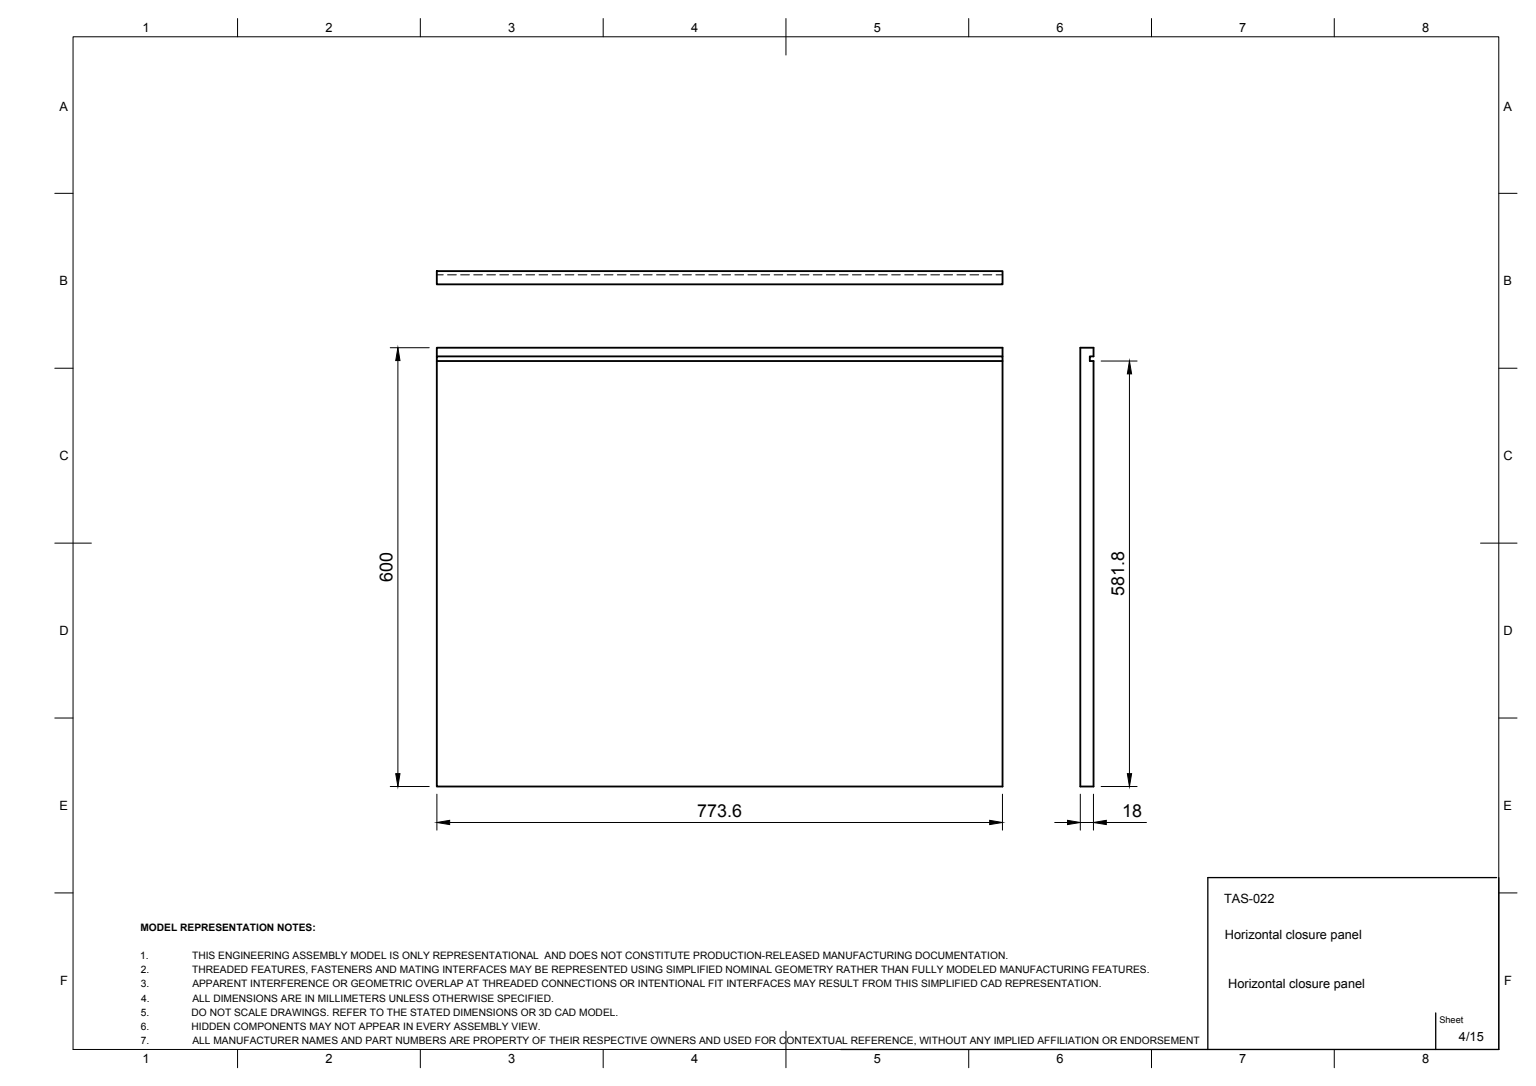
ISO-10303-21;
HEADER;
/* Generated by software containing ST-Developer
 * from STEP Tools, Inc. (www.steptools.com) 
 */

FILE_DESCRIPTION(
/* description */ (''),
/* implementation_level */ '2;1');

FILE_NAME(
/* name */ 'Horizontal closure panel.step',
/* time_stamp */ '2026-11-15T21:02:08-08:00',
/* author */ (''),
/* organization */ (''),
/* preprocessor_version */ 'ST-DEVELOPER v20.2',
/* originating_system */ 'Autodesk Translation Framework v15.17.0.0',
/* authorisation */ '');

FILE_SCHEMA (('AUTOMOTIVE_DESIGN { 1 0 10303 214 3 1 1 }'));
ENDSEC;

DATA;
#10=MECHANICAL_DESIGN_GEOMETRIC_PRESENTATION_REPRESENTATION('',(#609),#31566);
#579=SHAPE_REPRESENTATION_RELATIONSHIP('SRR','None',#31643,#594);
#594=ADVANCED_BREP_SHAPE_REPRESENTATION('',(#624),#31558);
#609=STYLED_ITEM('',(#31724),#624);
#624=MANIFOLD_SOLID_BREP('Body1',#5722);
#745=FACE_OUTER_BOUND('',#1042,.T.);
#746=FACE_OUTER_BOUND('',#1043,.T.);
#747=FACE_OUTER_BOUND('',#1044,.T.);
#748=FACE_OUTER_BOUND('',#1045,.T.);
#749=FACE_OUTER_BOUND('',#1046,.T.);
#750=FACE_OUTER_BOUND('',#1047,.T.);
#751=FACE_OUTER_BOUND('',#1048,.T.);
#752=FACE_OUTER_BOUND('',#1049,.T.);
#753=FACE_OUTER_BOUND('',#1050,.T.);
#754=FACE_OUTER_BOUND('',#1051,.T.);
#1042=EDGE_LOOP('',(#4197,#4198,#4199,#4200));
#1043=EDGE_LOOP('',(#4201,#4202,#4203,#4204));
#1044=EDGE_LOOP('',(#4205,#4206,#4207,#4208));
#1045=EDGE_LOOP('',(#4209,#4210,#4211,#4212,#4213,#4214,#4215,#4216));
#1046=EDGE_LOOP('',(#4217,#4218,#4219,#4220));
#1047=EDGE_LOOP('',(#4221,#4222,#4223,#4224));
#1048=EDGE_LOOP('',(#4225,#4226,#4227,#4228));
#1049=EDGE_LOOP('',(#4229,#4230,#4231,#4232,#4233,#4234,#4235,#4236));
#1050=EDGE_LOOP('',(#4237,#4238,#4239,#4240));
#1051=EDGE_LOOP('',(#4241,#4242,#4243,#4244));
#1439=LINE('',#8161,#1946);
#1440=LINE('',#8163,#1947);
#1441=LINE('',#8165,#1948);
#1442=LINE('',#8166,#1949);
#1443=LINE('',#8170,#1950);
#1444=LINE('',#8172,#1951);
#1445=LINE('',#8174,#1952);
#1446=LINE('',#8175,#1953);
#1447=LINE('',#8177,#1954);
#1448=LINE('',#8178,#1955);
#1449=LINE('',#8181,#1956);
#1450=LINE('',#8183,#1957);
#1451=LINE('',#8185,#1958);
#1452=LINE('',#8187,#1959);
#1453=LINE('',#8188,#1960);
#1454=LINE('',#8191,#1961);
#1455=LINE('',#8192,#1962);
#1456=LINE('',#8195,#1963);
#1457=LINE('',#8197,#1964);
#1458=LINE('',#8198,#1965);
#1459=LINE('',#8201,#1966);
#1460=LINE('',#8202,#1967);
#1461=LINE('',#8204,#1968);
#1462=LINE('',#8205,#1969);
#1946=VECTOR('',#6865,1.);
#1947=VECTOR('',#6866,1.);
#1948=VECTOR('',#6867,1.);
#1949=VECTOR('',#6868,1.);
#1950=VECTOR('',#6871,1.);
#1951=VECTOR('',#6872,1.);
#1952=VECTOR('',#6873,1.);
#1953=VECTOR('',#6874,1.);
#1954=VECTOR('',#6877,1.);
#1955=VECTOR('',#6878,1.);
#1956=VECTOR('',#6881,1.);
#1957=VECTOR('',#6882,1.);
#1958=VECTOR('',#6883,1.);
#1959=VECTOR('',#6884,1.);
#1960=VECTOR('',#6885,1.);
#1961=VECTOR('',#6888,1.);
#1962=VECTOR('',#6889,1.);
#1963=VECTOR('',#6892,1.);
#1964=VECTOR('',#6893,1.);
#1965=VECTOR('',#6894,1.);
#1966=VECTOR('',#6897,1.);
#1967=VECTOR('',#6898,1.);
#1968=VECTOR('',#6901,1.);
#1969=VECTOR('',#6902,1.);
#2410=VERTEX_POINT('',#8159);
#2411=VERTEX_POINT('',#8160);
#2412=VERTEX_POINT('',#8162);
#2413=VERTEX_POINT('',#8164);
#2414=VERTEX_POINT('',#8168);
#2415=VERTEX_POINT('',#8169);
#2416=VERTEX_POINT('',#8171);
#2417=VERTEX_POINT('',#8173);
#2418=VERTEX_POINT('',#8180);
#2419=VERTEX_POINT('',#8182);
#2420=VERTEX_POINT('',#8184);
#2421=VERTEX_POINT('',#8186);
#2422=VERTEX_POINT('',#8190);
#2423=VERTEX_POINT('',#8194);
#2424=VERTEX_POINT('',#8196);
#2425=VERTEX_POINT('',#8200);
#3094=EDGE_CURVE('',#2410,#2411,#1439,.T.);
#3095=EDGE_CURVE('',#2412,#2410,#1440,.T.);
#3096=EDGE_CURVE('',#2413,#2412,#1441,.T.);
#3097=EDGE_CURVE('',#2411,#2413,#1442,.T.);
#3098=EDGE_CURVE('',#2414,#2415,#1443,.T.);
#3099=EDGE_CURVE('',#2416,#2414,#1444,.T.);
#3100=EDGE_CURVE('',#2417,#2416,#1445,.T.);
#3101=EDGE_CURVE('',#2415,#2417,#1446,.T.);
#3102=EDGE_CURVE('',#2413,#2416,#1447,.T.);
#3103=EDGE_CURVE('',#2417,#2412,#1448,.T.);
#3104=EDGE_CURVE('',#2418,#2410,#1449,.T.);
#3105=EDGE_CURVE('',#2419,#2418,#1450,.T.);
#3106=EDGE_CURVE('',#2419,#2420,#1451,.T.);
#3107=EDGE_CURVE('',#2420,#2421,#1452,.T.);
#3108=EDGE_CURVE('',#2415,#2421,#1453,.T.);
#3109=EDGE_CURVE('',#2411,#2422,#1454,.T.);
#3110=EDGE_CURVE('',#2422,#2418,#1455,.T.);
#3111=EDGE_CURVE('',#2420,#2423,#1456,.T.);
#3112=EDGE_CURVE('',#2423,#2424,#1457,.T.);
#3113=EDGE_CURVE('',#2421,#2424,#1458,.T.);
#3114=EDGE_CURVE('',#2425,#2419,#1459,.T.);
#3115=EDGE_CURVE('',#2425,#2422,#1460,.T.);
#3116=EDGE_CURVE('',#2424,#2414,#1461,.T.);
#3117=EDGE_CURVE('',#2423,#2425,#1462,.T.);
#4197=ORIENTED_EDGE('',*,*,#3094,.F.);
#4198=ORIENTED_EDGE('',*,*,#3095,.F.);
#4199=ORIENTED_EDGE('',*,*,#3096,.F.);
#4200=ORIENTED_EDGE('',*,*,#3097,.F.);
#4201=ORIENTED_EDGE('',*,*,#3098,.F.);
#4202=ORIENTED_EDGE('',*,*,#3099,.F.);
#4203=ORIENTED_EDGE('',*,*,#3100,.F.);
#4204=ORIENTED_EDGE('',*,*,#3101,.F.);
#4205=ORIENTED_EDGE('',*,*,#3102,.F.);
#4206=ORIENTED_EDGE('',*,*,#3096,.T.);
#4207=ORIENTED_EDGE('',*,*,#3103,.F.);
#4208=ORIENTED_EDGE('',*,*,#3100,.T.);
#4209=ORIENTED_EDGE('',*,*,#3101,.T.);
#4210=ORIENTED_EDGE('',*,*,#3103,.T.);
#4211=ORIENTED_EDGE('',*,*,#3095,.T.);
#4212=ORIENTED_EDGE('',*,*,#3104,.F.);
#4213=ORIENTED_EDGE('',*,*,#3105,.F.);
#4214=ORIENTED_EDGE('',*,*,#3106,.T.);
#4215=ORIENTED_EDGE('',*,*,#3107,.T.);
#4216=ORIENTED_EDGE('',*,*,#3108,.F.);
#4217=ORIENTED_EDGE('',*,*,#3094,.T.);
#4218=ORIENTED_EDGE('',*,*,#3109,.T.);
#4219=ORIENTED_EDGE('',*,*,#3110,.T.);
#4220=ORIENTED_EDGE('',*,*,#3104,.T.);
#4221=ORIENTED_EDGE('',*,*,#3111,.T.);
#4222=ORIENTED_EDGE('',*,*,#3112,.T.);
#4223=ORIENTED_EDGE('',*,*,#3113,.F.);
#4224=ORIENTED_EDGE('',*,*,#3107,.F.);
#4225=ORIENTED_EDGE('',*,*,#3114,.T.);
#4226=ORIENTED_EDGE('',*,*,#3105,.T.);
#4227=ORIENTED_EDGE('',*,*,#3110,.F.);
#4228=ORIENTED_EDGE('',*,*,#3115,.F.);
#4229=ORIENTED_EDGE('',*,*,#3099,.T.);
#4230=ORIENTED_EDGE('',*,*,#3116,.F.);
#4231=ORIENTED_EDGE('',*,*,#3112,.F.);
#4232=ORIENTED_EDGE('',*,*,#3117,.T.);
#4233=ORIENTED_EDGE('',*,*,#3115,.T.);
#4234=ORIENTED_EDGE('',*,*,#3109,.F.);
#4235=ORIENTED_EDGE('',*,*,#3097,.T.);
#4236=ORIENTED_EDGE('',*,*,#3102,.T.);
#4237=ORIENTED_EDGE('',*,*,#3098,.T.);
#4238=ORIENTED_EDGE('',*,*,#3108,.T.);
#4239=ORIENTED_EDGE('',*,*,#3113,.T.);
#4240=ORIENTED_EDGE('',*,*,#3116,.T.);
#4241=ORIENTED_EDGE('',*,*,#3117,.F.);
#4242=ORIENTED_EDGE('',*,*,#3111,.F.);
#4243=ORIENTED_EDGE('',*,*,#3106,.F.);
#4244=ORIENTED_EDGE('',*,*,#3114,.F.);
#5350=PLANE('',#6070);
#5351=PLANE('',#6071);
#5352=PLANE('',#6072);
#5353=PLANE('',#6073);
#5354=PLANE('',#6074);
#5355=PLANE('',#6075);
#5356=PLANE('',#6076);
#5357=PLANE('',#6077);
#5358=PLANE('',#6078);
#5359=PLANE('',#6079);
#5559=ADVANCED_FACE('',(#745),#5350,.F.);
#5560=ADVANCED_FACE('',(#746),#5351,.F.);
#5561=ADVANCED_FACE('',(#747),#5352,.T.);
#5562=ADVANCED_FACE('',(#748),#5353,.T.);
#5563=ADVANCED_FACE('',(#749),#5354,.T.);
#5564=ADVANCED_FACE('',(#750),#5355,.T.);
#5565=ADVANCED_FACE('',(#751),#5356,.T.);
#5566=ADVANCED_FACE('',(#752),#5357,.T.);
#5567=ADVANCED_FACE('',(#753),#5358,.T.);
#5568=ADVANCED_FACE('',(#754),#5359,.F.);
#5722=CLOSED_SHELL('',(#5559,#5560,#5561,#5562,#5563,#5564,#5565,#5566,
#5567,#5568));
#6069=AXIS2_PLACEMENT_3D('',#8157,#6861,#6862);
#6070=AXIS2_PLACEMENT_3D('',#8158,#6863,#6864);
#6071=AXIS2_PLACEMENT_3D('',#8167,#6869,#6870);
#6072=AXIS2_PLACEMENT_3D('',#8176,#6875,#6876);
#6073=AXIS2_PLACEMENT_3D('',#8179,#6879,#6880);
#6074=AXIS2_PLACEMENT_3D('',#8189,#6886,#6887);
#6075=AXIS2_PLACEMENT_3D('',#8193,#6890,#6891);
#6076=AXIS2_PLACEMENT_3D('',#8199,#6895,#6896);
#6077=AXIS2_PLACEMENT_3D('',#8203,#6899,#6900);
#6078=AXIS2_PLACEMENT_3D('',#8206,#6903,#6904);
#6079=AXIS2_PLACEMENT_3D('',#8207,#6905,#6906);
#6861=DIRECTION('axis',(0.,0.,1.));
#6862=DIRECTION('refdir',(1.,0.,0.));
#6863=DIRECTION('center_axis',(0.,-1.,0.));
#6864=DIRECTION('ref_axis',(1.,0.,0.));
#6865=DIRECTION('',(-1.,0.,0.));
#6866=DIRECTION('',(0.,0.,1.));
#6867=DIRECTION('',(1.,0.,0.));
#6868=DIRECTION('',(0.,0.,-1.));
#6869=DIRECTION('center_axis',(0.,1.,0.));
#6870=DIRECTION('ref_axis',(-1.,0.,0.));
#6871=DIRECTION('',(1.,0.,0.));
#6872=DIRECTION('',(0.,0.,1.));
#6873=DIRECTION('',(-1.,0.,0.));
#6874=DIRECTION('',(0.,0.,-1.));
#6875=DIRECTION('center_axis',(0.,0.,1.));
#6876=DIRECTION('ref_axis',(1.,0.,0.));
#6877=DIRECTION('',(0.,1.,0.));
#6878=DIRECTION('',(0.,-1.,0.));
#6879=DIRECTION('center_axis',(1.,0.,0.));
#6880=DIRECTION('ref_axis',(0.,1.,0.));
#6881=DIRECTION('',(0.,1.,0.));
#6882=DIRECTION('',(0.,0.,1.));
#6883=DIRECTION('',(0.,1.,0.));
#6884=DIRECTION('',(0.,0.,1.));
#6885=DIRECTION('',(0.,1.,0.));
#6886=DIRECTION('center_axis',(0.,0.,1.));
#6887=DIRECTION('ref_axis',(1.,0.,0.));
#6888=DIRECTION('',(0.,-1.,0.));
#6889=DIRECTION('',(1.,0.,0.));
#6890=DIRECTION('center_axis',(0.,1.,0.));
#6891=DIRECTION('ref_axis',(-1.,0.,0.));
#6892=DIRECTION('',(-1.,0.,0.));
#6893=DIRECTION('',(0.,0.,1.));
#6894=DIRECTION('',(-1.,0.,0.));
#6895=DIRECTION('center_axis',(0.,-1.,0.));
#6896=DIRECTION('ref_axis',(1.,0.,0.));
#6897=DIRECTION('',(1.,0.,0.));
#6898=DIRECTION('',(0.,0.,1.));
#6899=DIRECTION('center_axis',(-1.,0.,0.));
#6900=DIRECTION('ref_axis',(0.,-1.,0.));
#6901=DIRECTION('',(0.,-1.,0.));
#6902=DIRECTION('',(0.,-1.,0.));
#6903=DIRECTION('center_axis',(0.,0.,1.));
#6904=DIRECTION('ref_axis',(1.,0.,0.));
#6905=DIRECTION('center_axis',(0.,0.,1.));
#6906=DIRECTION('ref_axis',(1.,0.,0.));
#8157=CARTESIAN_POINT('',(0.,0.,0.));
#8158=CARTESIAN_POINT('Origin',(0.,58.18,1.3));
#8159=CARTESIAN_POINT('',(77.36,58.18,1.8));
#8160=CARTESIAN_POINT('',(0.,58.18,1.8));
#8161=CARTESIAN_POINT('',(19.34,58.18,1.8));
#8162=CARTESIAN_POINT('',(77.36,58.18,1.3));
#8163=CARTESIAN_POINT('',(77.36,58.18,0.65));
#8164=CARTESIAN_POINT('',(0.,58.18,1.3));
#8165=CARTESIAN_POINT('',(0.,58.18,1.3));
#8166=CARTESIAN_POINT('',(0.,58.18,0.65));
#8167=CARTESIAN_POINT('Origin',(77.36,58.82,1.3));
#8168=CARTESIAN_POINT('',(0.,58.82,1.8));
#8169=CARTESIAN_POINT('',(77.36,58.82,1.8));
#8170=CARTESIAN_POINT('',(58.02,58.82,1.8));
#8171=CARTESIAN_POINT('',(0.,58.82,1.3));
#8172=CARTESIAN_POINT('',(0.,58.82,0.65));
#8173=CARTESIAN_POINT('',(77.36,58.82,1.3));
#8174=CARTESIAN_POINT('',(77.36,58.82,1.3));
#8175=CARTESIAN_POINT('',(77.36,58.82,0.65));
#8176=CARTESIAN_POINT('Origin',(38.68,58.5,1.3));
#8177=CARTESIAN_POINT('',(0.,59.25,1.3));
#8178=CARTESIAN_POINT('',(77.36,29.25,1.3));
#8179=CARTESIAN_POINT('Origin',(77.36,0.,0.));
#8180=CARTESIAN_POINT('',(77.36,0.,1.8));
#8181=CARTESIAN_POINT('',(77.36,0.,1.8));
#8182=CARTESIAN_POINT('',(77.36,0.,0.));
#8183=CARTESIAN_POINT('',(77.36,0.,0.));
#8184=CARTESIAN_POINT('',(77.36,60.,0.));
#8185=CARTESIAN_POINT('',(77.36,0.,0.));
#8186=CARTESIAN_POINT('',(77.36,60.,1.8));
#8187=CARTESIAN_POINT('',(77.36,60.,0.));
#8188=CARTESIAN_POINT('',(77.36,0.,1.8));
#8189=CARTESIAN_POINT('Origin',(38.68,30.,1.8));
#8190=CARTESIAN_POINT('',(0.,0.,1.8));
#8191=CARTESIAN_POINT('',(0.,60.,1.8));
#8192=CARTESIAN_POINT('',(0.,0.,1.8));
#8193=CARTESIAN_POINT('Origin',(77.36,60.,0.));
#8194=CARTESIAN_POINT('',(0.,60.,0.));
#8195=CARTESIAN_POINT('',(77.36,60.,0.));
#8196=CARTESIAN_POINT('',(0.,60.,1.8));
#8197=CARTESIAN_POINT('',(0.,60.,0.));
#8198=CARTESIAN_POINT('',(77.36,60.,1.8));
#8199=CARTESIAN_POINT('Origin',(0.,0.,0.));
#8200=CARTESIAN_POINT('',(0.,0.,0.));
#8201=CARTESIAN_POINT('',(0.,0.,0.));
#8202=CARTESIAN_POINT('',(0.,0.,0.));
#8203=CARTESIAN_POINT('Origin',(0.,60.,0.));
#8204=CARTESIAN_POINT('',(0.,60.,1.8));
#8205=CARTESIAN_POINT('',(0.,60.,0.));
#8206=CARTESIAN_POINT('Origin',(38.68,30.,1.8));
#8207=CARTESIAN_POINT('Origin',(38.68,30.,0.));
#31541=UNCERTAINTY_MEASURE_WITH_UNIT(LENGTH_MEASURE(0.001),#31567,
'DISTANCE_ACCURACY_VALUE',
'Maximum model space distance between geometric entities at asserted c
onnectivities');
#31549=UNCERTAINTY_MEASURE_WITH_UNIT(LENGTH_MEASURE(0.001),#31567,
'DISTANCE_ACCURACY_VALUE',
'Maximum model space distance between geometric entities at asserted c
onnectivities');
#31558=(
GEOMETRIC_REPRESENTATION_CONTEXT(3)
GLOBAL_UNCERTAINTY_ASSIGNED_CONTEXT((#31541))
GLOBAL_UNIT_ASSIGNED_CONTEXT((#31567,#31569,#31570))
REPRESENTATION_CONTEXT('','3D')
);
#31566=(
GEOMETRIC_REPRESENTATION_CONTEXT(3)
GLOBAL_UNCERTAINTY_ASSIGNED_CONTEXT((#31549))
GLOBAL_UNIT_ASSIGNED_CONTEXT((#31567,#31569,#31570))
REPRESENTATION_CONTEXT('','3D')
);
#31567=(
LENGTH_UNIT()
NAMED_UNIT(*)
SI_UNIT(.CENTI.,.METRE.)
);
#31569=(
NAMED_UNIT(*)
PLANE_ANGLE_UNIT()
SI_UNIT($,.RADIAN.)
);
#31570=(
NAMED_UNIT(*)
SI_UNIT($,.STERADIAN.)
SOLID_ANGLE_UNIT()
);
#31579=SHAPE_DEFINITION_REPRESENTATION(#31595,#31643);
#31595=PRODUCT_DEFINITION_SHAPE('',$,#31660);
#31643=SHAPE_REPRESENTATION('',(#6069),#31558);
#31651=PRODUCT_DEFINITION_CONTEXT('part definition',#31701,'design');
#31660=PRODUCT_DEFINITION('Horizontal closure panel',
'Horizontal closure panel',#31676,#31651);
#31676=PRODUCT_DEFINITION_FORMATION('',$,#31711);
#31701=APPLICATION_CONTEXT(
'Core Data for Automotive Mechanical Design Process');
#31702=PRODUCT_CONTEXT('part definition',#31701,'mechanical');
#31711=PRODUCT('Horizontal closure panel','Horizontal closure panel',$,
(#31702));
#31724=PRESENTATION_STYLE_ASSIGNMENT((#31731));
#31731=SURFACE_STYLE_USAGE(.BOTH.,#31738);
#31738=SURFACE_SIDE_STYLE('',(#31745));
#31745=SURFACE_STYLE_FILL_AREA(#31752);
#31752=FILL_AREA_STYLE('Opaque(169,210,234)',(#31759));
#31759=FILL_AREA_STYLE_COLOUR('Opaque(169,210,234)',#31766);
#31766=COLOUR_RGB('Opaque(169,210,234)',0.662745098039216,0.823529411764706,
0.917647058823529);
ENDSEC;
END-ISO-10303-21;
